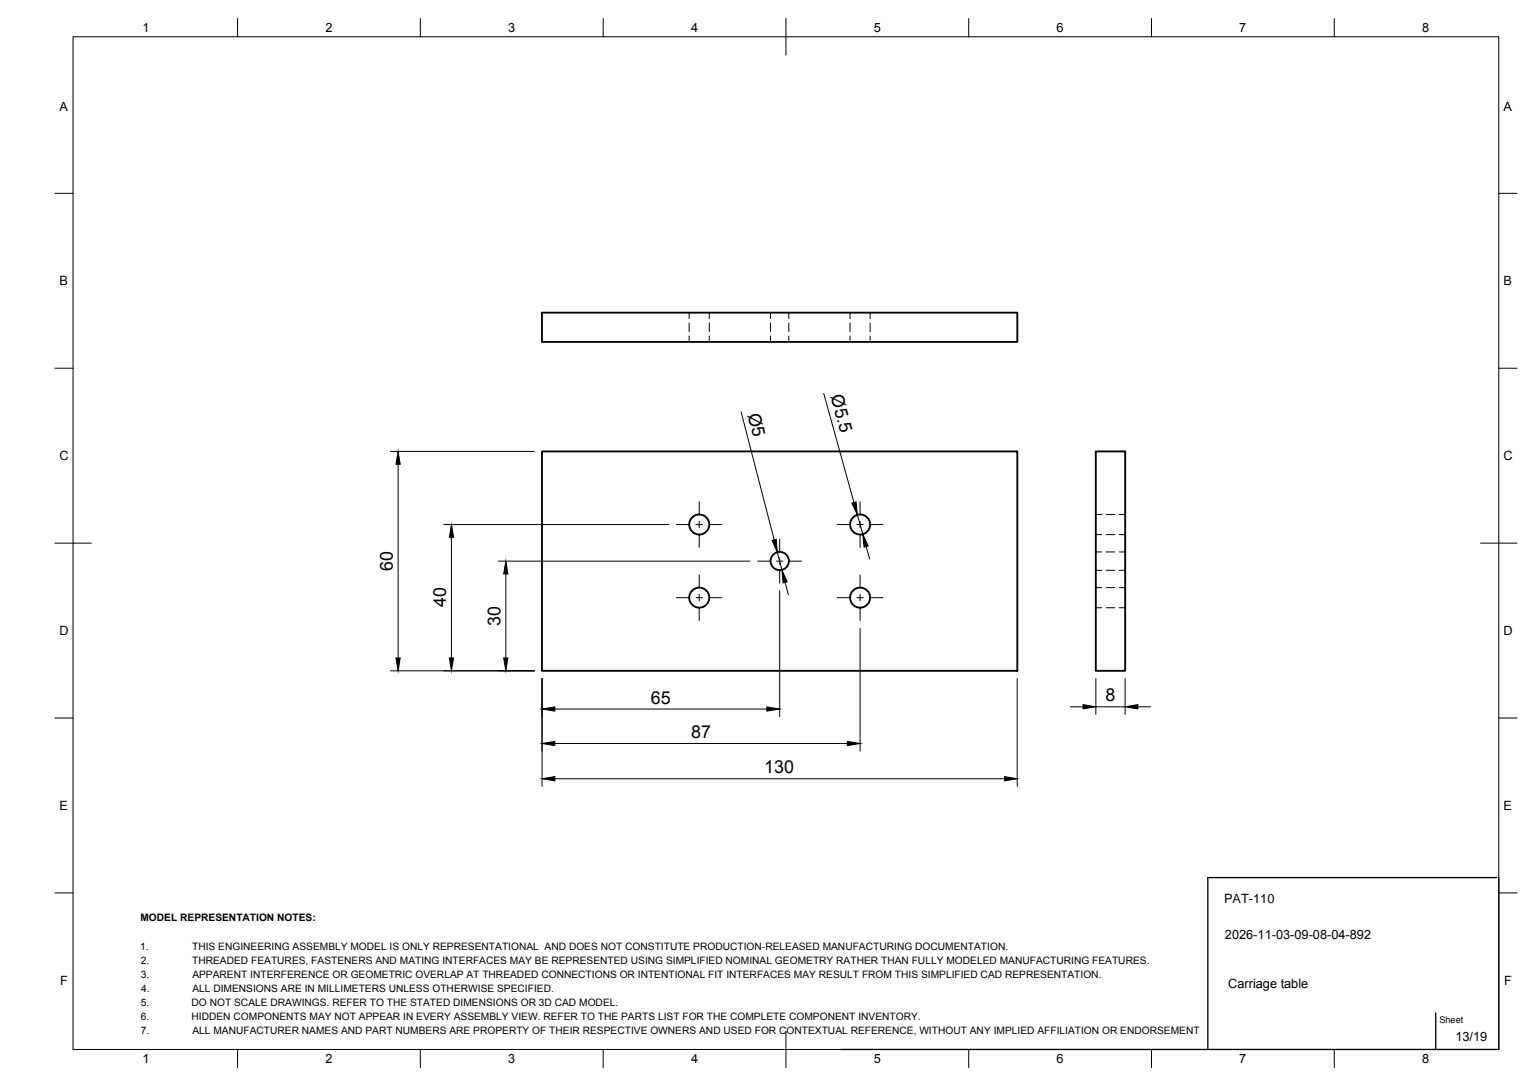
ISO-10303-21;
HEADER;
/* Generated by software containing ST-Developer
 * from STEP Tools, Inc. (www.steptools.com) 
 */

FILE_DESCRIPTION(
/* description */ ('Twin-shaft manual slide'),
/* implementation_level */ '2;1');

FILE_NAME(
/* name */ 'Carriage table.step',
/* time_stamp */ '2026-10-27T18:38:08-07:00',
/* author */ (''),
/* organization */ (''),
/* preprocessor_version */ 'ST-DEVELOPER v20.2',
/* originating_system */ 'Autodesk Translation Framework v15.17.0.0',
/* authorisation */ '');

FILE_SCHEMA (('AUTOMOTIVE_DESIGN { 1 0 10303 214 3 1 1 }'));
ENDSEC;

DATA;
#10=MECHANICAL_DESIGN_GEOMETRIC_PRESENTATION_REPRESENTATION('',(#283),#6463);
#251=SHAPE_REPRESENTATION_RELATIONSHIP('SRR','None',#6570,#267);
#267=ADVANCED_BREP_SHAPE_REPRESENTATION('',(#298),#6453);
#283=STYLED_ITEM('',(#6733),#298);
#298=MANIFOLD_SOLID_BREP('Body1',#3646);
#361=FACE_BOUND('',#900,.T.);
#362=FACE_BOUND('',#901,.T.);
#363=FACE_BOUND('',#902,.T.);
#364=FACE_BOUND('',#903,.T.);
#365=FACE_BOUND('',#904,.T.);
#366=FACE_BOUND('',#906,.T.);
#367=FACE_BOUND('',#907,.T.);
#368=FACE_BOUND('',#908,.T.);
#369=FACE_BOUND('',#909,.T.);
#370=FACE_BOUND('',#910,.T.);
#460=PLANE('',#4038);
#461=PLANE('',#4039);
#462=PLANE('',#4040);
#463=PLANE('',#4041);
#464=PLANE('',#4042);
#465=PLANE('',#4043);
#626=FACE_OUTER_BOUND('',#890,.T.);
#627=FACE_OUTER_BOUND('',#891,.T.);
#628=FACE_OUTER_BOUND('',#892,.T.);
#629=FACE_OUTER_BOUND('',#893,.T.);
#630=FACE_OUTER_BOUND('',#894,.T.);
#631=FACE_OUTER_BOUND('',#895,.T.);
#632=FACE_OUTER_BOUND('',#896,.T.);
#633=FACE_OUTER_BOUND('',#897,.T.);
#634=FACE_OUTER_BOUND('',#898,.T.);
#635=FACE_OUTER_BOUND('',#899,.T.);
#636=FACE_OUTER_BOUND('',#905,.T.);
#890=EDGE_LOOP('',(#2940,#2941,#2942,#2943));
#891=EDGE_LOOP('',(#2944,#2945,#2946,#2947));
#892=EDGE_LOOP('',(#2948,#2949,#2950,#2951));
#893=EDGE_LOOP('',(#2952,#2953,#2954,#2955));
#894=EDGE_LOOP('',(#2956,#2957,#2958,#2959));
#895=EDGE_LOOP('',(#2960,#2961,#2962,#2963));
#896=EDGE_LOOP('',(#2964,#2965,#2966,#2967));
#897=EDGE_LOOP('',(#2968,#2969,#2970,#2971));
#898=EDGE_LOOP('',(#2972,#2973,#2974,#2975));
#899=EDGE_LOOP('',(#2976,#2977,#2978,#2979));
#900=EDGE_LOOP('',(#2980));
#901=EDGE_LOOP('',(#2981));
#902=EDGE_LOOP('',(#2982));
#903=EDGE_LOOP('',(#2983));
#904=EDGE_LOOP('',(#2984));
#905=EDGE_LOOP('',(#2985,#2986,#2987,#2988));
#906=EDGE_LOOP('',(#2989));
#907=EDGE_LOOP('',(#2990));
#908=EDGE_LOOP('',(#2991));
#909=EDGE_LOOP('',(#2992));
#910=EDGE_LOOP('',(#2993));
#1186=LINE('',#5907,#1472);
#1187=LINE('',#5913,#1473);
#1188=LINE('',#5919,#1474);
#1189=LINE('',#5925,#1475);
#1190=LINE('',#5931,#1476);
#1191=LINE('',#5936,#1477);
#1192=LINE('',#5938,#1478);
#1193=LINE('',#5940,#1479);
#1194=LINE('',#5941,#1480);
#1195=LINE('',#5944,#1481);
#1196=LINE('',#5946,#1482);
#1197=LINE('',#5947,#1483);
#1198=LINE('',#5950,#1484);
#1199=LINE('',#5952,#1485);
#1200=LINE('',#5953,#1486);
#1201=LINE('',#5955,#1487);
#1202=LINE('',#5956,#1488);
#1472=VECTOR('',#4796,0.25);
#1473=VECTOR('',#4803,0.274999999999999);
#1474=VECTOR('',#4810,0.275);
#1475=VECTOR('',#4817,0.275);
#1476=VECTOR('',#4824,0.274999999999999);
#1477=VECTOR('',#4829,1.);
#1478=VECTOR('',#4830,1.);
#1479=VECTOR('',#4831,1.);
#1480=VECTOR('',#4832,1.);
#1481=VECTOR('',#4835,1.);
#1482=VECTOR('',#4836,1.);
#1483=VECTOR('',#4837,1.);
#1484=VECTOR('',#4840,1.);
#1485=VECTOR('',#4841,1.);
#1486=VECTOR('',#4842,1.);
#1487=VECTOR('',#4845,1.);
#1488=VECTOR('',#4846,1.);
#1686=CIRCLE('',#4024,0.25);
#1687=CIRCLE('',#4025,0.25);
#1688=CIRCLE('',#4027,0.274999999999999);
#1689=CIRCLE('',#4028,0.274999999999999);
#1690=CIRCLE('',#4030,0.275);
#1691=CIRCLE('',#4031,0.275);
#1692=CIRCLE('',#4033,0.275);
#1693=CIRCLE('',#4034,0.275);
#1694=CIRCLE('',#4036,0.274999999999999);
#1695=CIRCLE('',#4037,0.274999999999999);
#1911=VERTEX_POINT('',#5904);
#1912=VERTEX_POINT('',#5906);
#1913=VERTEX_POINT('',#5910);
#1914=VERTEX_POINT('',#5912);
#1915=VERTEX_POINT('',#5916);
#1916=VERTEX_POINT('',#5918);
#1917=VERTEX_POINT('',#5922);
#1918=VERTEX_POINT('',#5924);
#1919=VERTEX_POINT('',#5928);
#1920=VERTEX_POINT('',#5930);
#1921=VERTEX_POINT('',#5934);
#1922=VERTEX_POINT('',#5935);
#1923=VERTEX_POINT('',#5937);
#1924=VERTEX_POINT('',#5939);
#1925=VERTEX_POINT('',#5943);
#1926=VERTEX_POINT('',#5945);
#1927=VERTEX_POINT('',#5949);
#1928=VERTEX_POINT('',#5951);
#2275=EDGE_CURVE('',#1911,#1911,#1686,.T.);
#2276=EDGE_CURVE('',#1911,#1912,#1186,.T.);
#2277=EDGE_CURVE('',#1912,#1912,#1687,.T.);
#2278=EDGE_CURVE('',#1913,#1913,#1688,.T.);
#2279=EDGE_CURVE('',#1913,#1914,#1187,.T.);
#2280=EDGE_CURVE('',#1914,#1914,#1689,.T.);
#2281=EDGE_CURVE('',#1915,#1915,#1690,.T.);
#2282=EDGE_CURVE('',#1915,#1916,#1188,.T.);
#2283=EDGE_CURVE('',#1916,#1916,#1691,.T.);
#2284=EDGE_CURVE('',#1917,#1917,#1692,.T.);
#2285=EDGE_CURVE('',#1917,#1918,#1189,.T.);
#2286=EDGE_CURVE('',#1918,#1918,#1693,.T.);
#2287=EDGE_CURVE('',#1919,#1919,#1694,.T.);
#2288=EDGE_CURVE('',#1919,#1920,#1190,.T.);
#2289=EDGE_CURVE('',#1920,#1920,#1695,.T.);
#2290=EDGE_CURVE('',#1921,#1922,#1191,.T.);
#2291=EDGE_CURVE('',#1922,#1923,#1192,.T.);
#2292=EDGE_CURVE('',#1924,#1923,#1193,.T.);
#2293=EDGE_CURVE('',#1921,#1924,#1194,.T.);
#2294=EDGE_CURVE('',#1925,#1921,#1195,.T.);
#2295=EDGE_CURVE('',#1926,#1924,#1196,.T.);
#2296=EDGE_CURVE('',#1925,#1926,#1197,.T.);
#2297=EDGE_CURVE('',#1927,#1925,#1198,.T.);
#2298=EDGE_CURVE('',#1928,#1926,#1199,.T.);
#2299=EDGE_CURVE('',#1927,#1928,#1200,.T.);
#2300=EDGE_CURVE('',#1922,#1927,#1201,.T.);
#2301=EDGE_CURVE('',#1923,#1928,#1202,.T.);
#2940=ORIENTED_EDGE('',*,*,#2275,.F.);
#2941=ORIENTED_EDGE('',*,*,#2276,.T.);
#2942=ORIENTED_EDGE('',*,*,#2277,.F.);
#2943=ORIENTED_EDGE('',*,*,#2276,.F.);
#2944=ORIENTED_EDGE('',*,*,#2278,.F.);
#2945=ORIENTED_EDGE('',*,*,#2279,.T.);
#2946=ORIENTED_EDGE('',*,*,#2280,.F.);
#2947=ORIENTED_EDGE('',*,*,#2279,.F.);
#2948=ORIENTED_EDGE('',*,*,#2281,.F.);
#2949=ORIENTED_EDGE('',*,*,#2282,.T.);
#2950=ORIENTED_EDGE('',*,*,#2283,.F.);
#2951=ORIENTED_EDGE('',*,*,#2282,.F.);
#2952=ORIENTED_EDGE('',*,*,#2284,.F.);
#2953=ORIENTED_EDGE('',*,*,#2285,.T.);
#2954=ORIENTED_EDGE('',*,*,#2286,.F.);
#2955=ORIENTED_EDGE('',*,*,#2285,.F.);
#2956=ORIENTED_EDGE('',*,*,#2287,.F.);
#2957=ORIENTED_EDGE('',*,*,#2288,.T.);
#2958=ORIENTED_EDGE('',*,*,#2289,.F.);
#2959=ORIENTED_EDGE('',*,*,#2288,.F.);
#2960=ORIENTED_EDGE('',*,*,#2290,.T.);
#2961=ORIENTED_EDGE('',*,*,#2291,.T.);
#2962=ORIENTED_EDGE('',*,*,#2292,.F.);
#2963=ORIENTED_EDGE('',*,*,#2293,.F.);
#2964=ORIENTED_EDGE('',*,*,#2294,.T.);
#2965=ORIENTED_EDGE('',*,*,#2293,.T.);
#2966=ORIENTED_EDGE('',*,*,#2295,.F.);
#2967=ORIENTED_EDGE('',*,*,#2296,.F.);
#2968=ORIENTED_EDGE('',*,*,#2297,.T.);
#2969=ORIENTED_EDGE('',*,*,#2296,.T.);
#2970=ORIENTED_EDGE('',*,*,#2298,.F.);
#2971=ORIENTED_EDGE('',*,*,#2299,.F.);
#2972=ORIENTED_EDGE('',*,*,#2300,.T.);
#2973=ORIENTED_EDGE('',*,*,#2299,.T.);
#2974=ORIENTED_EDGE('',*,*,#2301,.F.);
#2975=ORIENTED_EDGE('',*,*,#2291,.F.);
#2976=ORIENTED_EDGE('',*,*,#2301,.T.);
#2977=ORIENTED_EDGE('',*,*,#2298,.T.);
#2978=ORIENTED_EDGE('',*,*,#2295,.T.);
#2979=ORIENTED_EDGE('',*,*,#2292,.T.);
#2980=ORIENTED_EDGE('',*,*,#2277,.T.);
#2981=ORIENTED_EDGE('',*,*,#2280,.T.);
#2982=ORIENTED_EDGE('',*,*,#2283,.T.);
#2983=ORIENTED_EDGE('',*,*,#2286,.T.);
#2984=ORIENTED_EDGE('',*,*,#2289,.T.);
#2985=ORIENTED_EDGE('',*,*,#2300,.F.);
#2986=ORIENTED_EDGE('',*,*,#2290,.F.);
#2987=ORIENTED_EDGE('',*,*,#2294,.F.);
#2988=ORIENTED_EDGE('',*,*,#2297,.F.);
#2989=ORIENTED_EDGE('',*,*,#2275,.T.);
#2990=ORIENTED_EDGE('',*,*,#2278,.T.);
#2991=ORIENTED_EDGE('',*,*,#2281,.T.);
#2992=ORIENTED_EDGE('',*,*,#2284,.T.);
#2993=ORIENTED_EDGE('',*,*,#2287,.T.);
#3402=CYLINDRICAL_SURFACE('',#4023,0.25);
#3403=CYLINDRICAL_SURFACE('',#4026,0.274999999999999);
#3404=CYLINDRICAL_SURFACE('',#4029,0.275);
#3405=CYLINDRICAL_SURFACE('',#4032,0.275);
#3406=CYLINDRICAL_SURFACE('',#4035,0.274999999999999);
#3531=ADVANCED_FACE('',(#626),#3402,.F.);
#3532=ADVANCED_FACE('',(#627),#3403,.F.);
#3533=ADVANCED_FACE('',(#628),#3404,.F.);
#3534=ADVANCED_FACE('',(#629),#3405,.F.);
#3535=ADVANCED_FACE('',(#630),#3406,.F.);
#3536=ADVANCED_FACE('',(#631),#460,.T.);
#3537=ADVANCED_FACE('',(#632),#461,.T.);
#3538=ADVANCED_FACE('',(#633),#462,.T.);
#3539=ADVANCED_FACE('',(#634),#463,.T.);
#3540=ADVANCED_FACE('',(#635,#361,#362,#363,#364,#365),#464,.T.);
#3541=ADVANCED_FACE('',(#636,#366,#367,#368,#369,#370),#465,.F.);
#3646=CLOSED_SHELL('',(#3531,#3532,#3533,#3534,#3535,#3536,#3537,#3538,
#3539,#3540,#3541));
#4022=AXIS2_PLACEMENT_3D('',#5902,#4790,#4791);
#4023=AXIS2_PLACEMENT_3D('',#5903,#4792,#4793);
#4024=AXIS2_PLACEMENT_3D('',#5905,#4794,#4795);
#4025=AXIS2_PLACEMENT_3D('',#5908,#4797,#4798);
#4026=AXIS2_PLACEMENT_3D('',#5909,#4799,#4800);
#4027=AXIS2_PLACEMENT_3D('',#5911,#4801,#4802);
#4028=AXIS2_PLACEMENT_3D('',#5914,#4804,#4805);
#4029=AXIS2_PLACEMENT_3D('',#5915,#4806,#4807);
#4030=AXIS2_PLACEMENT_3D('',#5917,#4808,#4809);
#4031=AXIS2_PLACEMENT_3D('',#5920,#4811,#4812);
#4032=AXIS2_PLACEMENT_3D('',#5921,#4813,#4814);
#4033=AXIS2_PLACEMENT_3D('',#5923,#4815,#4816);
#4034=AXIS2_PLACEMENT_3D('',#5926,#4818,#4819);
#4035=AXIS2_PLACEMENT_3D('',#5927,#4820,#4821);
#4036=AXIS2_PLACEMENT_3D('',#5929,#4822,#4823);
#4037=AXIS2_PLACEMENT_3D('',#5932,#4825,#4826);
#4038=AXIS2_PLACEMENT_3D('',#5933,#4827,#4828);
#4039=AXIS2_PLACEMENT_3D('',#5942,#4833,#4834);
#4040=AXIS2_PLACEMENT_3D('',#5948,#4838,#4839);
#4041=AXIS2_PLACEMENT_3D('',#5954,#4843,#4844);
#4042=AXIS2_PLACEMENT_3D('',#5957,#4847,#4848);
#4043=AXIS2_PLACEMENT_3D('',#5958,#4849,#4850);
#4790=DIRECTION('axis',(0.,0.,1.));
#4791=DIRECTION('refdir',(1.,0.,0.));
#4792=DIRECTION('center_axis',(0.,0.,1.));
#4793=DIRECTION('ref_axis',(1.,0.,0.));
#4794=DIRECTION('center_axis',(0.,0.,1.));
#4795=DIRECTION('ref_axis',(1.,0.,0.));
#4796=DIRECTION('',(0.,0.,1.));
#4797=DIRECTION('center_axis',(0.,0.,-1.));
#4798=DIRECTION('ref_axis',(1.,0.,0.));
#4799=DIRECTION('center_axis',(0.,0.,1.));
#4800=DIRECTION('ref_axis',(1.,0.,0.));
#4801=DIRECTION('center_axis',(0.,0.,1.));
#4802=DIRECTION('ref_axis',(1.,0.,0.));
#4803=DIRECTION('',(0.,0.,1.));
#4804=DIRECTION('center_axis',(0.,0.,-1.));
#4805=DIRECTION('ref_axis',(1.,0.,0.));
#4806=DIRECTION('center_axis',(0.,0.,1.));
#4807=DIRECTION('ref_axis',(1.,0.,0.));
#4808=DIRECTION('center_axis',(0.,0.,1.));
#4809=DIRECTION('ref_axis',(1.,0.,0.));
#4810=DIRECTION('',(0.,0.,1.));
#4811=DIRECTION('center_axis',(0.,0.,-1.));
#4812=DIRECTION('ref_axis',(1.,0.,0.));
#4813=DIRECTION('center_axis',(0.,0.,1.));
#4814=DIRECTION('ref_axis',(1.,0.,0.));
#4815=DIRECTION('center_axis',(0.,0.,1.));
#4816=DIRECTION('ref_axis',(1.,0.,0.));
#4817=DIRECTION('',(0.,0.,1.));
#4818=DIRECTION('center_axis',(0.,0.,-1.));
#4819=DIRECTION('ref_axis',(1.,0.,0.));
#4820=DIRECTION('center_axis',(0.,0.,1.));
#4821=DIRECTION('ref_axis',(1.,0.,0.));
#4822=DIRECTION('center_axis',(0.,0.,1.));
#4823=DIRECTION('ref_axis',(1.,0.,0.));
#4824=DIRECTION('',(0.,0.,1.));
#4825=DIRECTION('center_axis',(0.,0.,-1.));
#4826=DIRECTION('ref_axis',(1.,0.,0.));
#4827=DIRECTION('center_axis',(0.,1.,0.));
#4828=DIRECTION('ref_axis',(-1.,0.,0.));
#4829=DIRECTION('',(-1.,0.,0.));
#4830=DIRECTION('',(0.,0.,1.));
#4831=DIRECTION('',(-1.,0.,0.));
#4832=DIRECTION('',(0.,0.,1.));
#4833=DIRECTION('center_axis',(1.,0.,0.));
#4834=DIRECTION('ref_axis',(0.,1.,0.));
#4835=DIRECTION('',(0.,1.,0.));
#4836=DIRECTION('',(0.,1.,0.));
#4837=DIRECTION('',(0.,0.,1.));
#4838=DIRECTION('center_axis',(0.,-1.,0.));
#4839=DIRECTION('ref_axis',(1.,0.,0.));
#4840=DIRECTION('',(1.,0.,0.));
#4841=DIRECTION('',(1.,0.,0.));
#4842=DIRECTION('',(0.,0.,1.));
#4843=DIRECTION('center_axis',(-1.,0.,0.));
#4844=DIRECTION('ref_axis',(0.,-1.,0.));
#4845=DIRECTION('',(0.,-1.,0.));
#4846=DIRECTION('',(0.,-1.,0.));
#4847=DIRECTION('center_axis',(0.,0.,1.));
#4848=DIRECTION('ref_axis',(1.,0.,0.));
#4849=DIRECTION('center_axis',(0.,0.,1.));
#4850=DIRECTION('ref_axis',(1.,0.,0.));
#5902=CARTESIAN_POINT('',(0.,0.,0.));
#5903=CARTESIAN_POINT('Origin',(15.,0.,5.7));
#5904=CARTESIAN_POINT('',(14.75,-3.06161699786838E-17,5.8));
#5905=CARTESIAN_POINT('Origin',(15.,0.,5.8));
#5906=CARTESIAN_POINT('',(14.75,3.06161699786838E-17,6.6));
#5907=CARTESIAN_POINT('',(14.75,-3.06161699786838E-17,5.7));
#5908=CARTESIAN_POINT('Origin',(15.,0.,6.6));
#5909=CARTESIAN_POINT('Origin',(16.,-2.2,5.7));
#5910=CARTESIAN_POINT('',(15.725,-2.2,5.8));
#5911=CARTESIAN_POINT('Origin',(16.,-2.2,5.8));
#5912=CARTESIAN_POINT('',(15.725,-2.2,6.6));
#5913=CARTESIAN_POINT('',(15.725,-2.2,5.7));
#5914=CARTESIAN_POINT('Origin',(16.,-2.2,6.6));
#5915=CARTESIAN_POINT('Origin',(14.,2.2,5.7));
#5916=CARTESIAN_POINT('',(13.725,2.2,5.8));
#5917=CARTESIAN_POINT('Origin',(14.,2.2,5.8));
#5918=CARTESIAN_POINT('',(13.725,2.2,6.6));
#5919=CARTESIAN_POINT('',(13.725,2.2,5.7));
#5920=CARTESIAN_POINT('Origin',(14.,2.2,6.6));
#5921=CARTESIAN_POINT('Origin',(14.,-2.2,5.7));
#5922=CARTESIAN_POINT('',(13.725,-2.2,5.8));
#5923=CARTESIAN_POINT('Origin',(14.,-2.2,5.8));
#5924=CARTESIAN_POINT('',(13.725,-2.2,6.6));
#5925=CARTESIAN_POINT('',(13.725,-2.2,5.7));
#5926=CARTESIAN_POINT('Origin',(14.,-2.2,6.6));
#5927=CARTESIAN_POINT('Origin',(16.,2.2,5.7));
#5928=CARTESIAN_POINT('',(15.725,2.2,5.8));
#5929=CARTESIAN_POINT('Origin',(16.,2.2,5.8));
#5930=CARTESIAN_POINT('',(15.725,2.2,6.6));
#5931=CARTESIAN_POINT('',(15.725,2.2,5.7));
#5932=CARTESIAN_POINT('Origin',(16.,2.2,6.6));
#5933=CARTESIAN_POINT('Origin',(18.,6.5,5.8));
#5934=CARTESIAN_POINT('',(18.,6.5,5.8));
#5935=CARTESIAN_POINT('',(12.,6.5,5.8));
#5936=CARTESIAN_POINT('',(18.,6.5,5.8));
#5937=CARTESIAN_POINT('',(12.,6.5,6.6));
#5938=CARTESIAN_POINT('',(12.,6.5,5.8));
#5939=CARTESIAN_POINT('',(18.,6.5,6.6));
#5940=CARTESIAN_POINT('',(18.,6.5,6.6));
#5941=CARTESIAN_POINT('',(18.,6.5,5.8));
#5942=CARTESIAN_POINT('Origin',(18.,-6.5,5.8));
#5943=CARTESIAN_POINT('',(18.,-6.5,5.8));
#5944=CARTESIAN_POINT('',(18.,-6.5,5.8));
#5945=CARTESIAN_POINT('',(18.,-6.5,6.6));
#5946=CARTESIAN_POINT('',(18.,-6.5,6.6));
#5947=CARTESIAN_POINT('',(18.,-6.5,5.8));
#5948=CARTESIAN_POINT('Origin',(12.,-6.5,5.8));
#5949=CARTESIAN_POINT('',(12.,-6.5,5.8));
#5950=CARTESIAN_POINT('',(12.,-6.5,5.8));
#5951=CARTESIAN_POINT('',(12.,-6.5,6.6));
#5952=CARTESIAN_POINT('',(12.,-6.5,6.6));
#5953=CARTESIAN_POINT('',(12.,-6.5,5.8));
#5954=CARTESIAN_POINT('Origin',(12.,6.5,5.8));
#5955=CARTESIAN_POINT('',(12.,6.5,5.8));
#5956=CARTESIAN_POINT('',(12.,6.5,6.6));
#5957=CARTESIAN_POINT('Origin',(15.,0.,6.6));
#5958=CARTESIAN_POINT('Origin',(15.,0.,5.8));
#6432=UNCERTAINTY_MEASURE_WITH_UNIT(LENGTH_MEASURE(0.001),#6464,
'DISTANCE_ACCURACY_VALUE',
'Maximum model space distance between geometric entities at asserted c
onnectivities');
#6442=UNCERTAINTY_MEASURE_WITH_UNIT(LENGTH_MEASURE(0.001),#6464,
'DISTANCE_ACCURACY_VALUE',
'Maximum model space distance between geometric entities at asserted c
onnectivities');
#6453=(
GEOMETRIC_REPRESENTATION_CONTEXT(3)
GLOBAL_UNCERTAINTY_ASSIGNED_CONTEXT((#6432))
GLOBAL_UNIT_ASSIGNED_CONTEXT((#6464,#6466,#6467))
REPRESENTATION_CONTEXT('','3D')
);
#6463=(
GEOMETRIC_REPRESENTATION_CONTEXT(3)
GLOBAL_UNCERTAINTY_ASSIGNED_CONTEXT((#6442))
GLOBAL_UNIT_ASSIGNED_CONTEXT((#6464,#6466,#6467))
REPRESENTATION_CONTEXT('','3D')
);
#6464=(
LENGTH_UNIT()
NAMED_UNIT(*)
SI_UNIT(.CENTI.,.METRE.)
);
#6466=(
NAMED_UNIT(*)
PLANE_ANGLE_UNIT()
SI_UNIT($,.RADIAN.)
);
#6467=(
NAMED_UNIT(*)
SI_UNIT($,.STERADIAN.)
SOLID_ANGLE_UNIT()
);
#6478=SHAPE_DEFINITION_REPRESENTATION(#6498,#6570);
#6498=PRODUCT_DEFINITION_SHAPE('',$,#6591);
#6570=SHAPE_REPRESENTATION('',(#4022),#6453);
#6580=PRODUCT_DEFINITION_CONTEXT('part definition',#6642,'design');
#6591=PRODUCT_DEFINITION('Carriage table','Carriage table',#6611,#6580);
#6611=PRODUCT_DEFINITION_FORMATION('',$,#6654);
#6642=APPLICATION_CONTEXT(
'Core Data for Automotive Mechanical Design Process');
#6643=PRODUCT_CONTEXT('part definition',#6642,'mechanical');
#6654=PRODUCT('Carriage table','Carriage table','Carriage table',(#6643));
#6727=COLOUR_RGB('Sky Blue',0.24,0.69,0.87);
#6728=FILL_AREA_STYLE_COLOUR('',#6727);
#6729=FILL_AREA_STYLE('',(#6728));
#6730=SURFACE_STYLE_FILL_AREA(#6729);
#6731=SURFACE_SIDE_STYLE('',(#6730));
#6732=SURFACE_STYLE_USAGE(.BOTH.,#6731);
#6733=PRESENTATION_STYLE_ASSIGNMENT((#6732));
ENDSEC;
END-ISO-10303-21;
